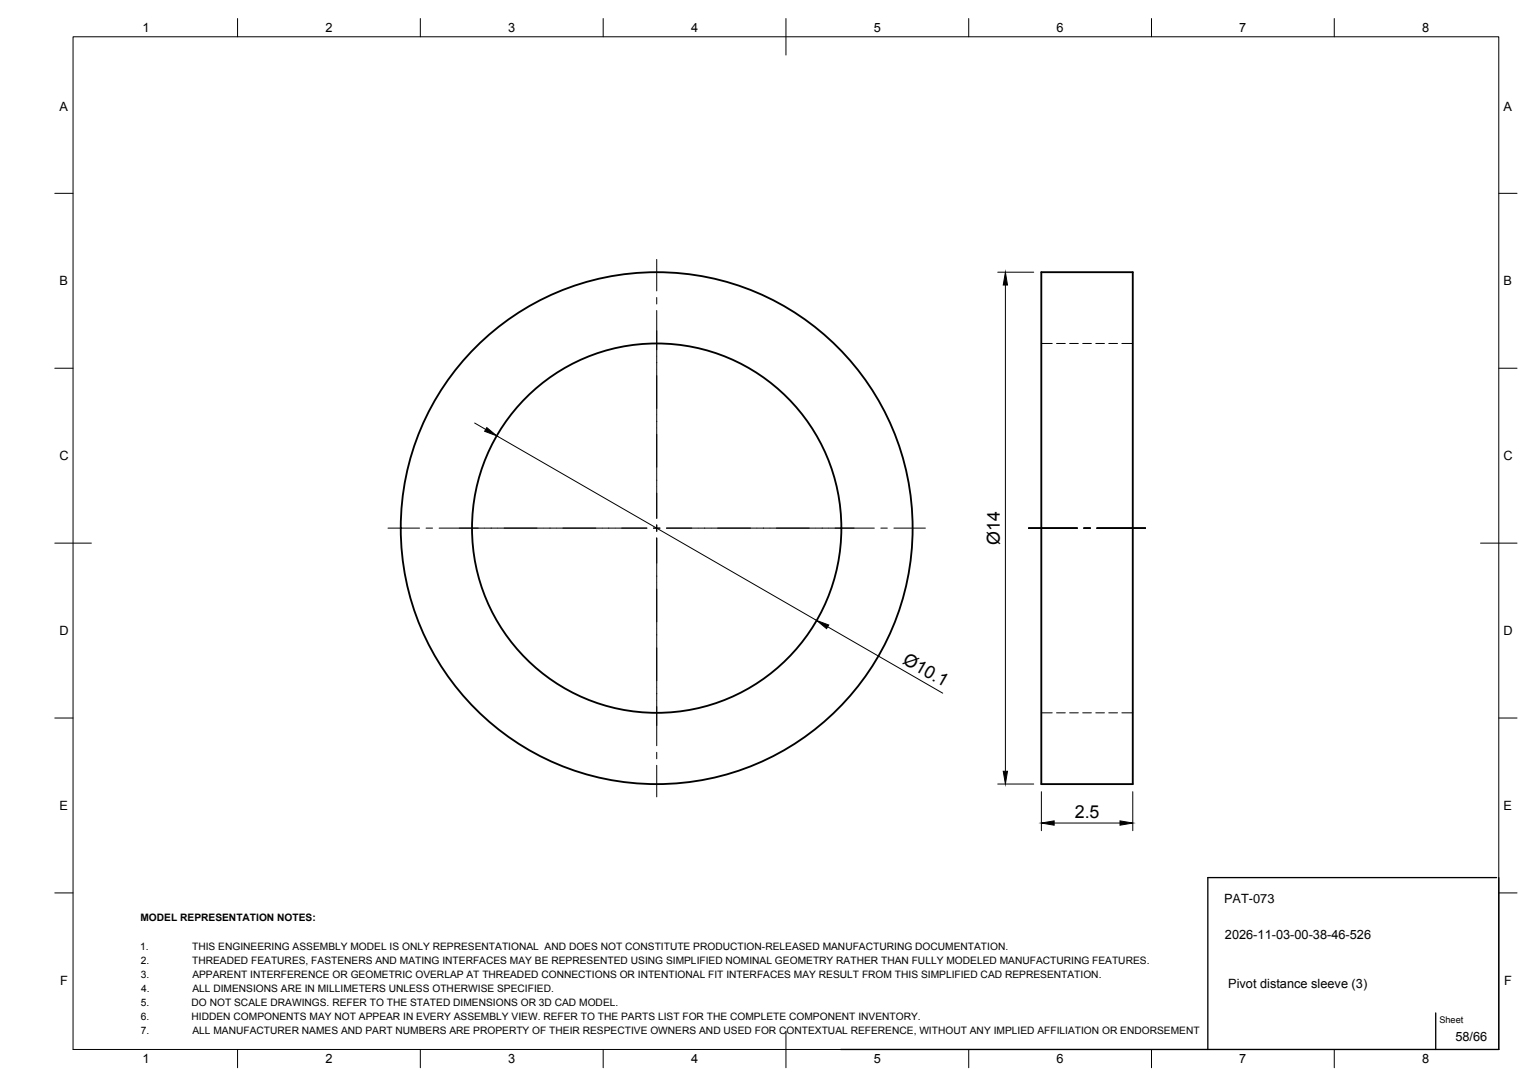
ISO-10303-21;
HEADER;
/* Generated by software containing ST-Developer
 * from STEP Tools, Inc. (www.steptools.com) 
 */

FILE_DESCRIPTION(
/* description */ ('Manual piston pump'),
/* implementation_level */ '2;1');

FILE_NAME(
/* name */ 'Pivot distance sleeve (3).step',
/* time_stamp */ '2026-11-02T16:54:23-08:00',
/* author */ (''),
/* organization */ (''),
/* preprocessor_version */ 'ST-DEVELOPER v20.2',
/* originating_system */ 'Autodesk Translation Framework v15.17.0.0',
/* authorisation */ '');

FILE_SCHEMA (('AUTOMOTIVE_DESIGN { 1 0 10303 214 3 1 1 }'));
ENDSEC;

DATA;
#10=MECHANICAL_DESIGN_GEOMETRIC_PRESENTATION_REPRESENTATION('',(#748),#19043);
#614=SHAPE_REPRESENTATION_RELATIONSHIP('SRR','None',#19364,#677);
#677=ADVANCED_BREP_SHAPE_REPRESENTATION('',(#816),#19031);
#748=STYLED_ITEM('',(#19664),#816);
#816=MANIFOLD_SOLID_BREP('Body1',#9536);
#1026=FACE_BOUND('',#2555,.T.);
#1027=FACE_BOUND('',#2557,.T.);
#1263=CYLINDRICAL_SURFACE('',#11301,0.505000000000001);
#1264=CYLINDRICAL_SURFACE('',#11304,0.699999999999999);
#1778=FACE_OUTER_BOUND('',#2552,.T.);
#1779=FACE_OUTER_BOUND('',#2553,.T.);
#1780=FACE_OUTER_BOUND('',#2554,.T.);
#1781=FACE_OUTER_BOUND('',#2556,.T.);
#2552=EDGE_LOOP('',(#8209,#8210,#8211,#8212));
#2553=EDGE_LOOP('',(#8213,#8214,#8215,#8216));
#2554=EDGE_LOOP('',(#8217));
#2555=EDGE_LOOP('',(#8218));
#2556=EDGE_LOOP('',(#8219));
#2557=EDGE_LOOP('',(#8220));
#3084=CIRCLE('',#11302,0.505000000000001);
#3085=CIRCLE('',#11303,0.505000000000001);
#3086=CIRCLE('',#11305,0.699999999999999);
#3087=CIRCLE('',#11306,0.699999999999999);
#3646=LINE('',#18364,#4250);
#3647=LINE('',#18370,#4251);
#4250=VECTOR('',#14114,0.505000000000001);
#4251=VECTOR('',#14121,0.699999999999999);
#5004=VERTEX_POINT('',#18361);
#5005=VERTEX_POINT('',#18363);
#5006=VERTEX_POINT('',#18367);
#5007=VERTEX_POINT('',#18369);
#6091=EDGE_CURVE('',#5004,#5004,#3084,.T.);
#6092=EDGE_CURVE('',#5004,#5005,#3646,.T.);
#6093=EDGE_CURVE('',#5005,#5005,#3085,.T.);
#6094=EDGE_CURVE('',#5006,#5006,#3086,.T.);
#6095=EDGE_CURVE('',#5006,#5007,#3647,.T.);
#6096=EDGE_CURVE('',#5007,#5007,#3087,.T.);
#8209=ORIENTED_EDGE('',*,*,#6091,.F.);
#8210=ORIENTED_EDGE('',*,*,#6092,.T.);
#8211=ORIENTED_EDGE('',*,*,#6093,.T.);
#8212=ORIENTED_EDGE('',*,*,#6092,.F.);
#8213=ORIENTED_EDGE('',*,*,#6094,.F.);
#8214=ORIENTED_EDGE('',*,*,#6095,.T.);
#8215=ORIENTED_EDGE('',*,*,#6096,.T.);
#8216=ORIENTED_EDGE('',*,*,#6095,.F.);
#8217=ORIENTED_EDGE('',*,*,#6094,.T.);
#8218=ORIENTED_EDGE('',*,*,#6091,.T.);
#8219=ORIENTED_EDGE('',*,*,#6096,.F.);
#8220=ORIENTED_EDGE('',*,*,#6093,.F.);
#8842=PLANE('',#11307);
#8843=PLANE('',#11308);
#9383=ADVANCED_FACE('',(#1778),#1263,.F.);
#9384=ADVANCED_FACE('',(#1779),#1264,.T.);
#9385=ADVANCED_FACE('',(#1780,#1026),#8842,.T.);
#9386=ADVANCED_FACE('',(#1781,#1027),#8843,.F.);
#9536=CLOSED_SHELL('',(#9383,#9384,#9385,#9386));
#11300=AXIS2_PLACEMENT_3D('',#18359,#14108,#14109);
#11301=AXIS2_PLACEMENT_3D('',#18360,#14110,#14111);
#11302=AXIS2_PLACEMENT_3D('',#18362,#14112,#14113);
#11303=AXIS2_PLACEMENT_3D('',#18365,#14115,#14116);
#11304=AXIS2_PLACEMENT_3D('',#18366,#14117,#14118);
#11305=AXIS2_PLACEMENT_3D('',#18368,#14119,#14120);
#11306=AXIS2_PLACEMENT_3D('',#18371,#14122,#14123);
#11307=AXIS2_PLACEMENT_3D('',#18372,#14124,#14125);
#11308=AXIS2_PLACEMENT_3D('',#18373,#14126,#14127);
#14108=DIRECTION('axis',(0.,0.,1.));
#14109=DIRECTION('refdir',(1.,0.,0.));
#14110=DIRECTION('center_axis',(1.,0.,0.));
#14111=DIRECTION('ref_axis',(0.,0.,-1.));
#14112=DIRECTION('center_axis',(-1.,0.,0.));
#14113=DIRECTION('ref_axis',(0.,0.,-1.));
#14114=DIRECTION('',(-1.,0.,0.));
#14115=DIRECTION('center_axis',(-1.,0.,0.));
#14116=DIRECTION('ref_axis',(0.,0.,-1.));
#14117=DIRECTION('center_axis',(1.,0.,0.));
#14118=DIRECTION('ref_axis',(0.,0.,-1.));
#14119=DIRECTION('center_axis',(1.,0.,0.));
#14120=DIRECTION('ref_axis',(0.,0.,-1.));
#14121=DIRECTION('',(-1.,0.,0.));
#14122=DIRECTION('center_axis',(1.,0.,0.));
#14123=DIRECTION('ref_axis',(0.,0.,-1.));
#14124=DIRECTION('center_axis',(1.,0.,0.));
#14125=DIRECTION('ref_axis',(0.,0.,-1.));
#14126=DIRECTION('center_axis',(1.,0.,0.));
#14127=DIRECTION('ref_axis',(0.,0.,-1.));
#18359=CARTESIAN_POINT('',(0.,0.,0.));
#18360=CARTESIAN_POINT('Origin',(3.95,-4.,10.));
#18361=CARTESIAN_POINT('',(4.2,-4.,10.505));
#18362=CARTESIAN_POINT('Origin',(4.2,-4.,10.));
#18363=CARTESIAN_POINT('',(3.95,-4.,10.505));
#18364=CARTESIAN_POINT('',(3.95,-4.,10.505));
#18365=CARTESIAN_POINT('Origin',(3.95,-4.,10.));
#18366=CARTESIAN_POINT('Origin',(3.95,-4.,10.));
#18367=CARTESIAN_POINT('',(4.2,-4.,10.7));
#18368=CARTESIAN_POINT('Origin',(4.2,-4.,10.));
#18369=CARTESIAN_POINT('',(3.95,-4.,10.7));
#18370=CARTESIAN_POINT('',(3.95,-4.,10.7));
#18371=CARTESIAN_POINT('Origin',(3.95,-4.,10.));
#18372=CARTESIAN_POINT('Origin',(4.2,-4.,10.));
#18373=CARTESIAN_POINT('Origin',(3.95,-4.,10.));
#18960=UNCERTAINTY_MEASURE_WITH_UNIT(LENGTH_MEASURE(0.001),#19044,
'DISTANCE_ACCURACY_VALUE',
'Maximum model space distance between geometric entities at asserted c
onnectivities');
#18972=UNCERTAINTY_MEASURE_WITH_UNIT(LENGTH_MEASURE(0.001),#19044,
'DISTANCE_ACCURACY_VALUE',
'Maximum model space distance between geometric entities at asserted c
onnectivities');
#19031=(
GEOMETRIC_REPRESENTATION_CONTEXT(3)
GLOBAL_UNCERTAINTY_ASSIGNED_CONTEXT((#18960))
GLOBAL_UNIT_ASSIGNED_CONTEXT((#19044,#19046,#19047))
REPRESENTATION_CONTEXT('','3D')
);
#19043=(
GEOMETRIC_REPRESENTATION_CONTEXT(3)
GLOBAL_UNCERTAINTY_ASSIGNED_CONTEXT((#18972))
GLOBAL_UNIT_ASSIGNED_CONTEXT((#19044,#19046,#19047))
REPRESENTATION_CONTEXT('','3D')
);
#19044=(
LENGTH_UNIT()
NAMED_UNIT(*)
SI_UNIT(.CENTI.,.METRE.)
);
#19046=(
NAMED_UNIT(*)
PLANE_ANGLE_UNIT()
SI_UNIT($,.RADIAN.)
);
#19047=(
NAMED_UNIT(*)
SI_UNIT($,.STERADIAN.)
SOLID_ANGLE_UNIT()
);
#19106=SHAPE_DEFINITION_REPRESENTATION(#19263,#19364);
#19263=PRODUCT_DEFINITION_SHAPE('',$,#19435);
#19364=SHAPE_REPRESENTATION('',(#11300),#19031);
#19376=PRODUCT_DEFINITION_CONTEXT('part definition',#19588,'design');
#19435=PRODUCT_DEFINITION('2026-11-03-00-38-46-526',
'Pivot distance sleeve (3)',#19505,#19376);
#19505=PRODUCT_DEFINITION_FORMATION('',$,#19648);
#19588=APPLICATION_CONTEXT(
'Core Data for Automotive Mechanical Design Process');
#19589=PRODUCT_CONTEXT('part definition',#19588,'mechanical');
#19648=PRODUCT('2026-11-03-00-38-46-526','Pivot distance sleeve (3)',
'Pivot distance sleeve',(#19589));
#19664=PRESENTATION_STYLE_ASSIGNMENT((#19670));
#19670=SURFACE_STYLE_USAGE(.BOTH.,#19676);
#19676=SURFACE_SIDE_STYLE('',(#19682));
#19682=SURFACE_STYLE_FILL_AREA(#19688);
#19688=FILL_AREA_STYLE('CAD Library Painted - Steel gray',(#19694));
#19694=FILL_AREA_STYLE_COLOUR('CAD Library Painted - Steel gray',#19700);
#19700=COLOUR_RGB('CAD Library Painted - Steel gray',0.592156862745098,
0.631372549019608,0.67843137254902);
ENDSEC;
END-ISO-10303-21;
